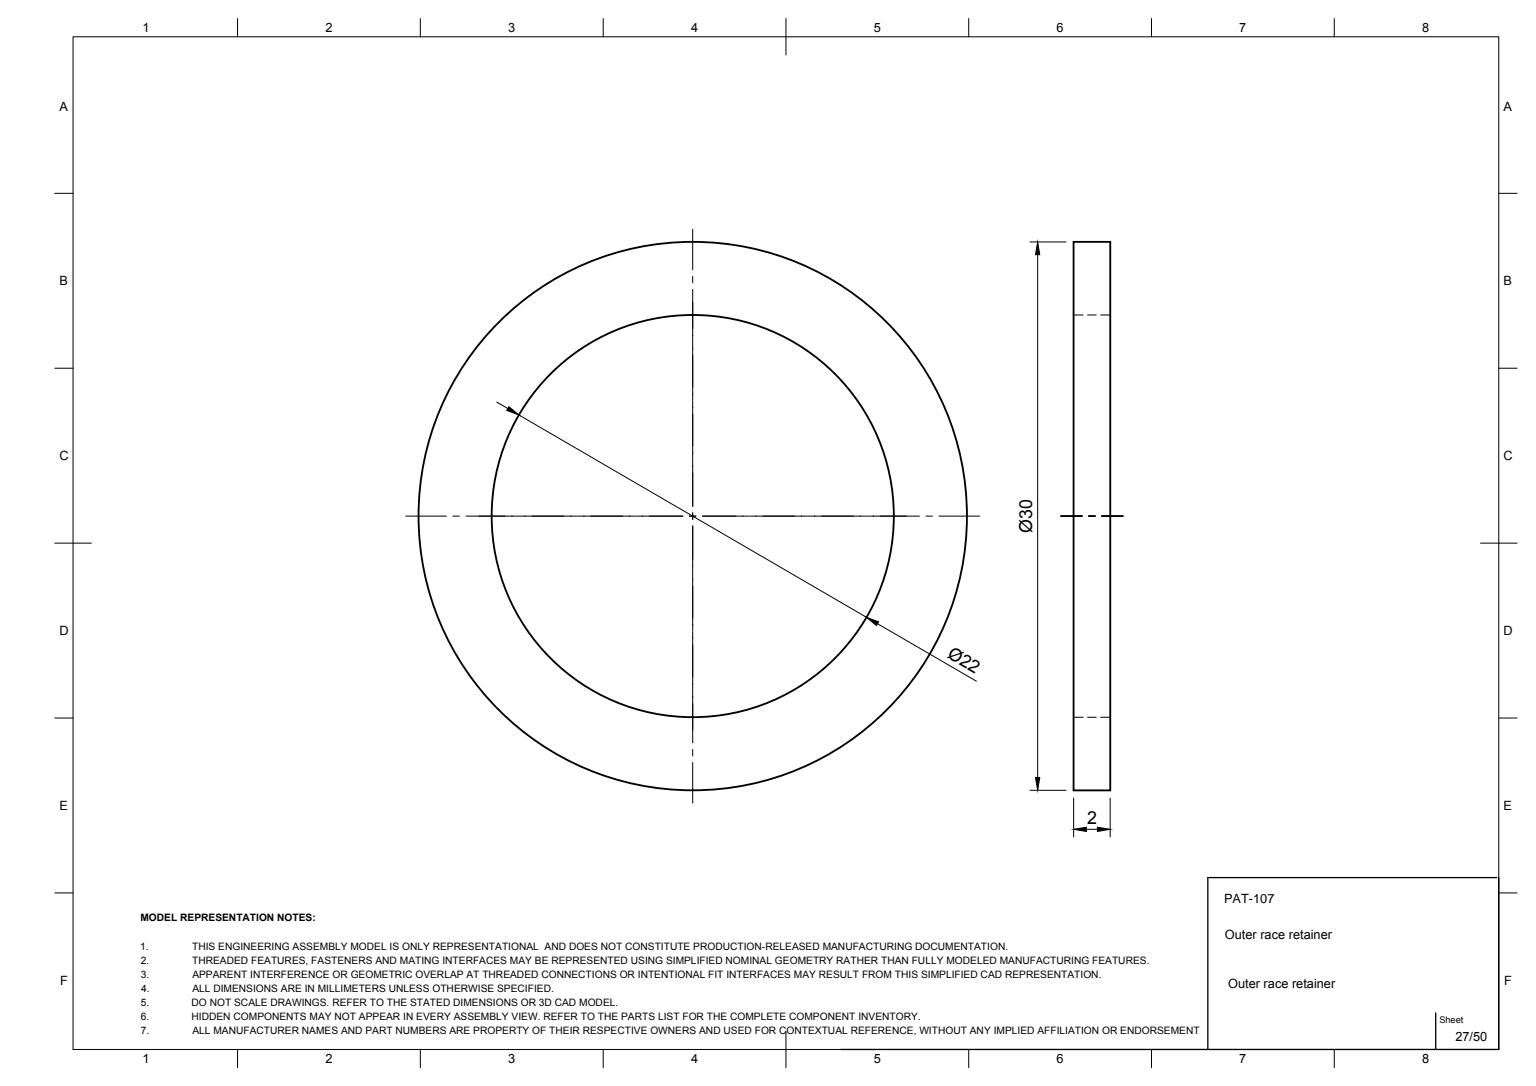
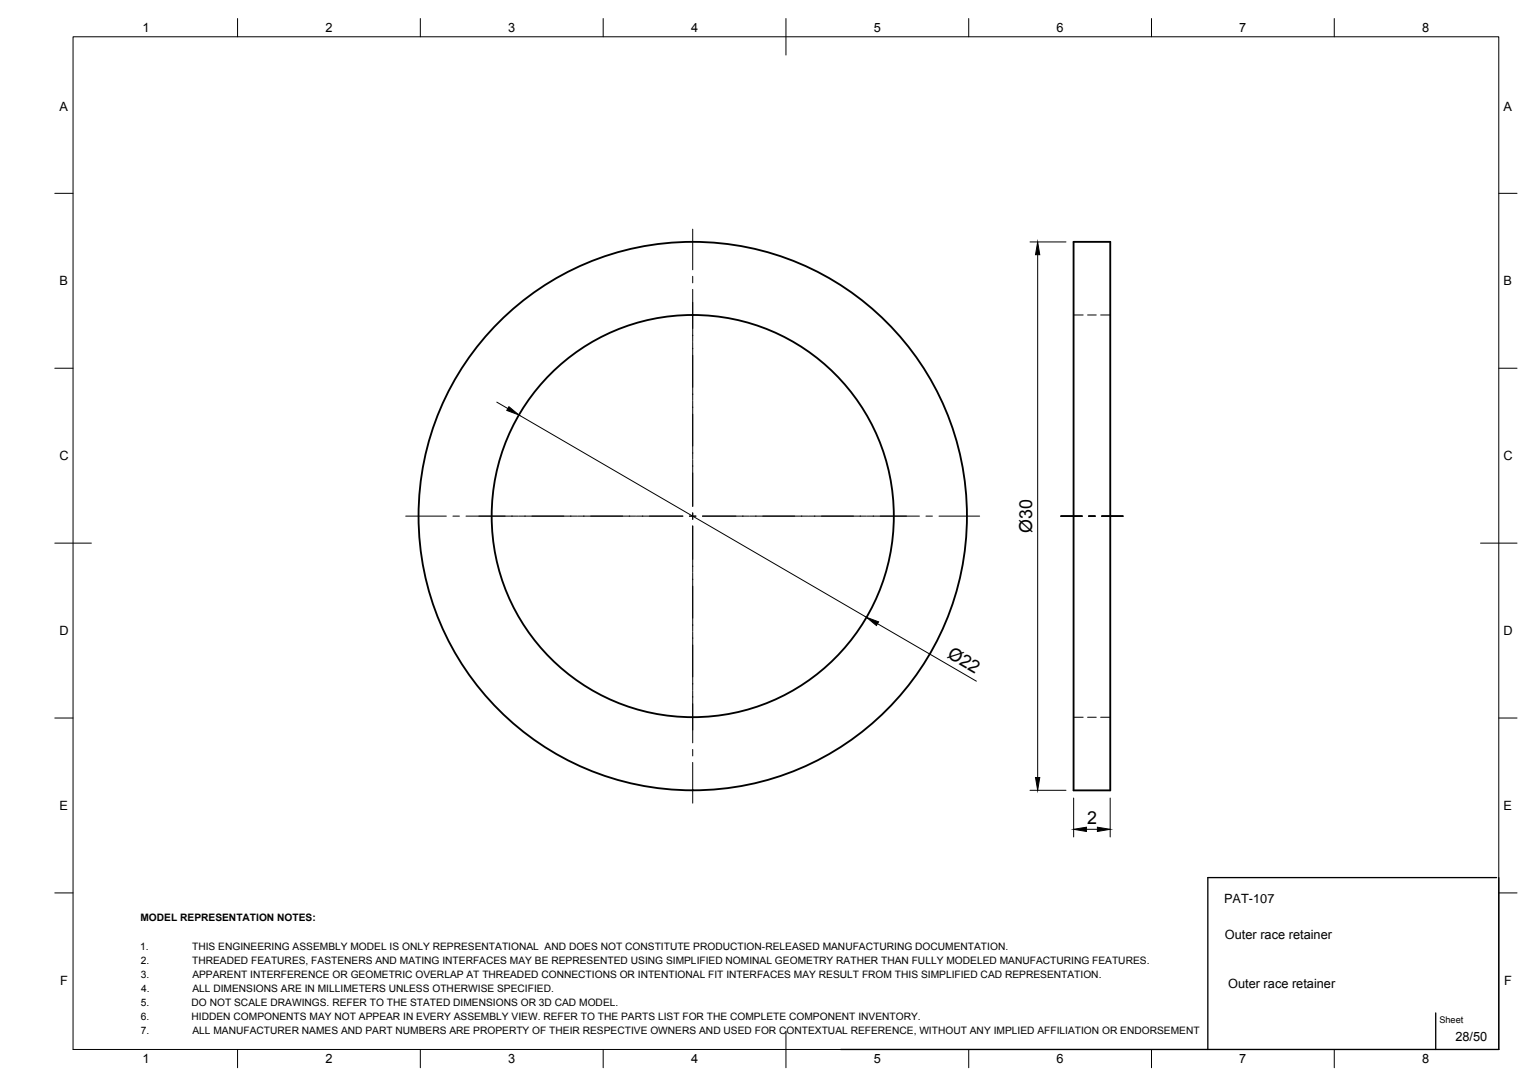
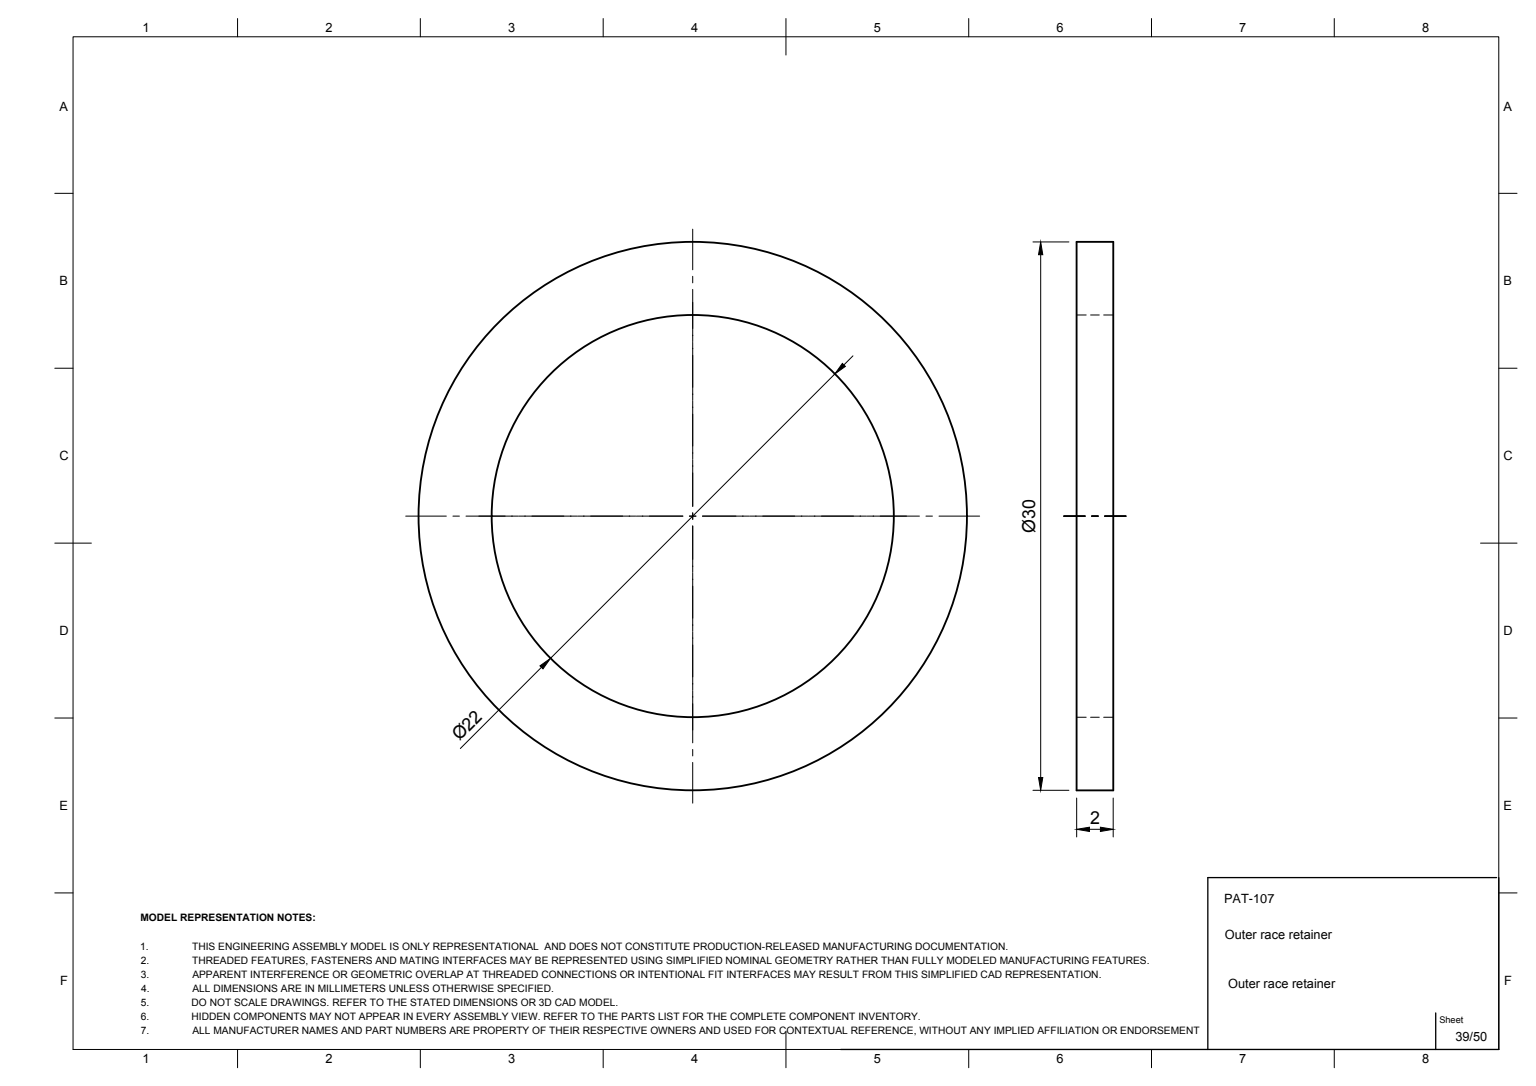
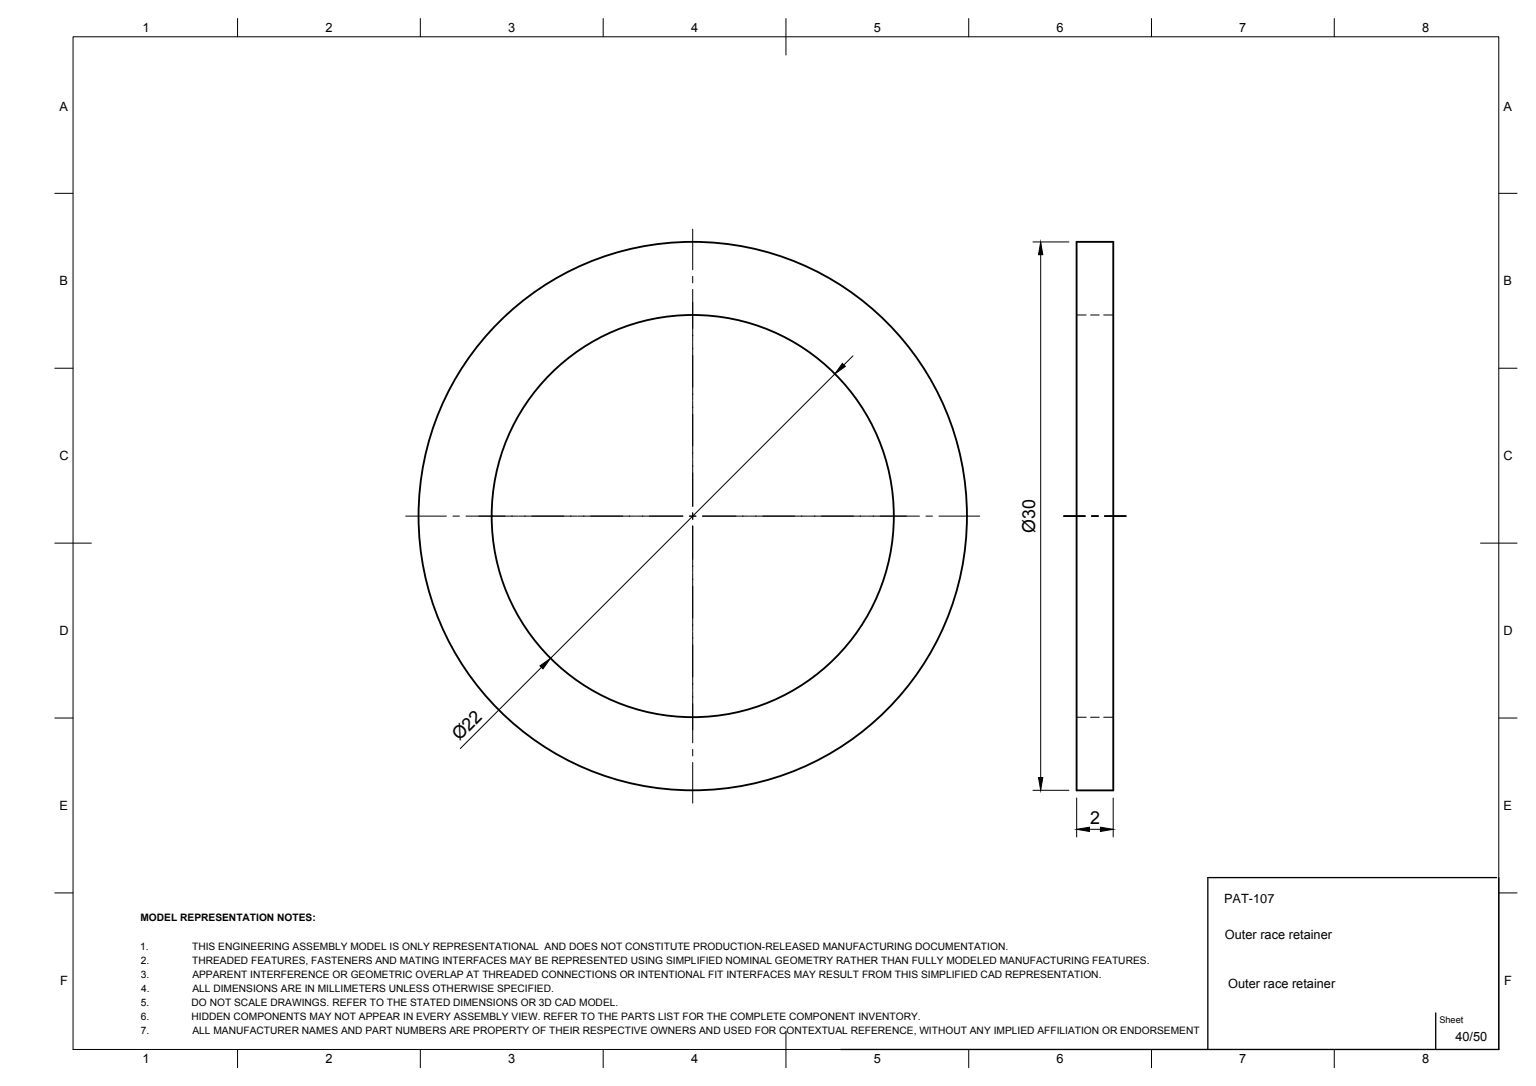
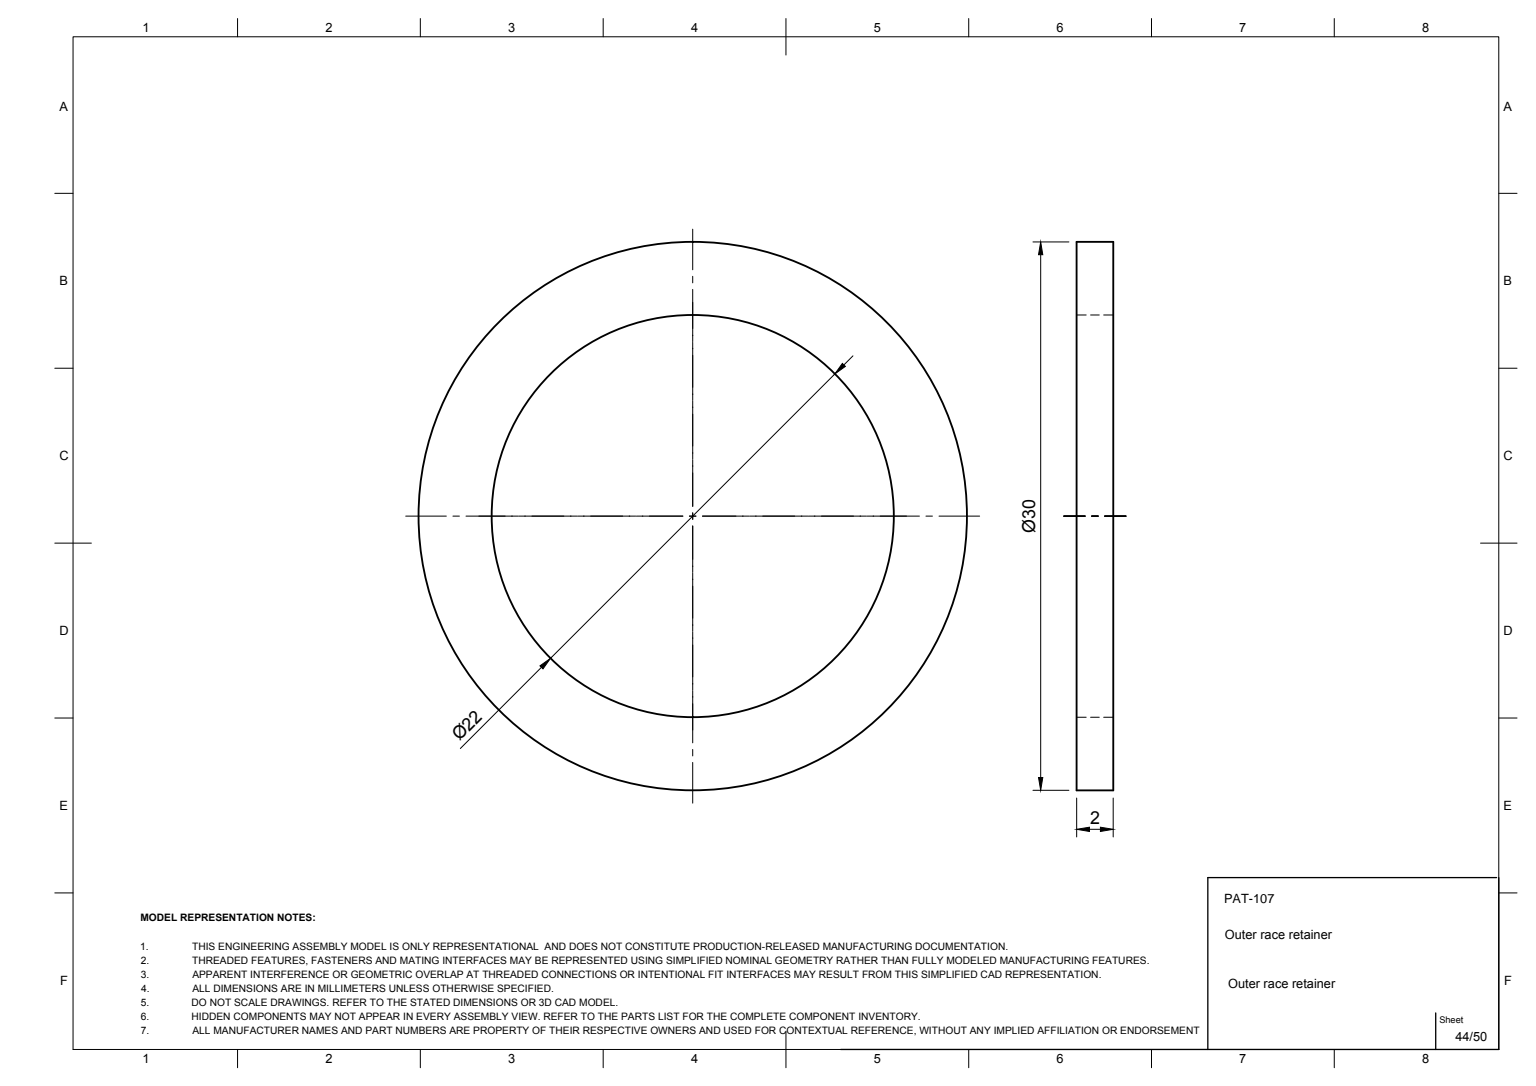
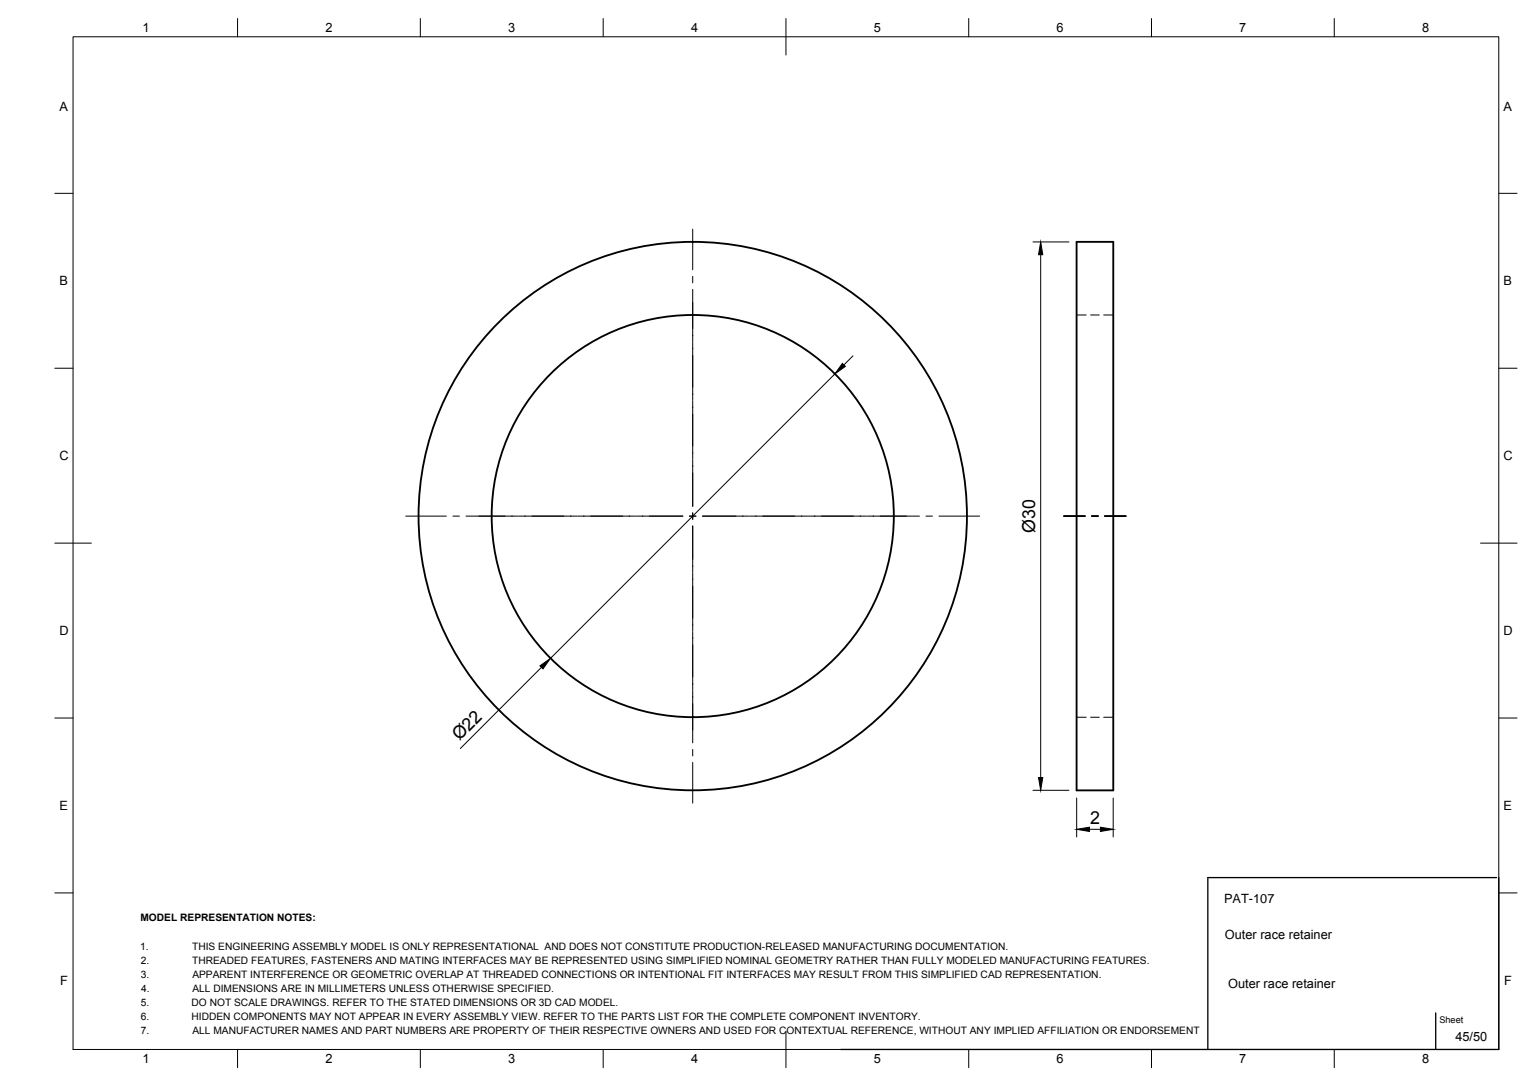
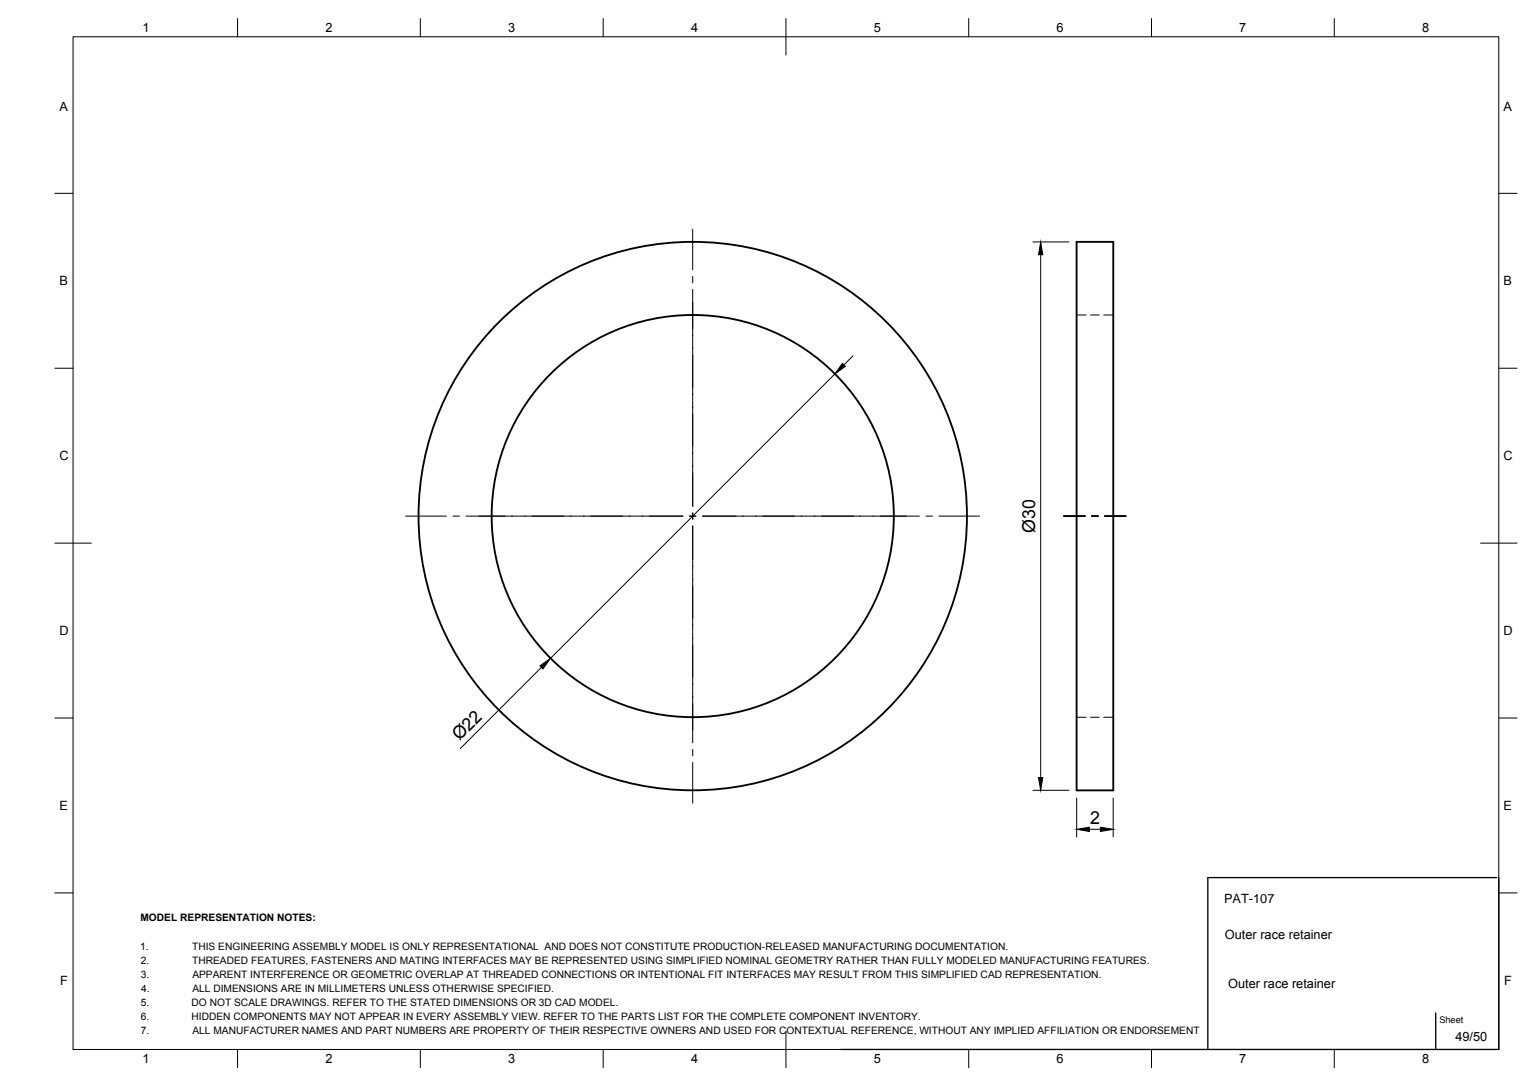
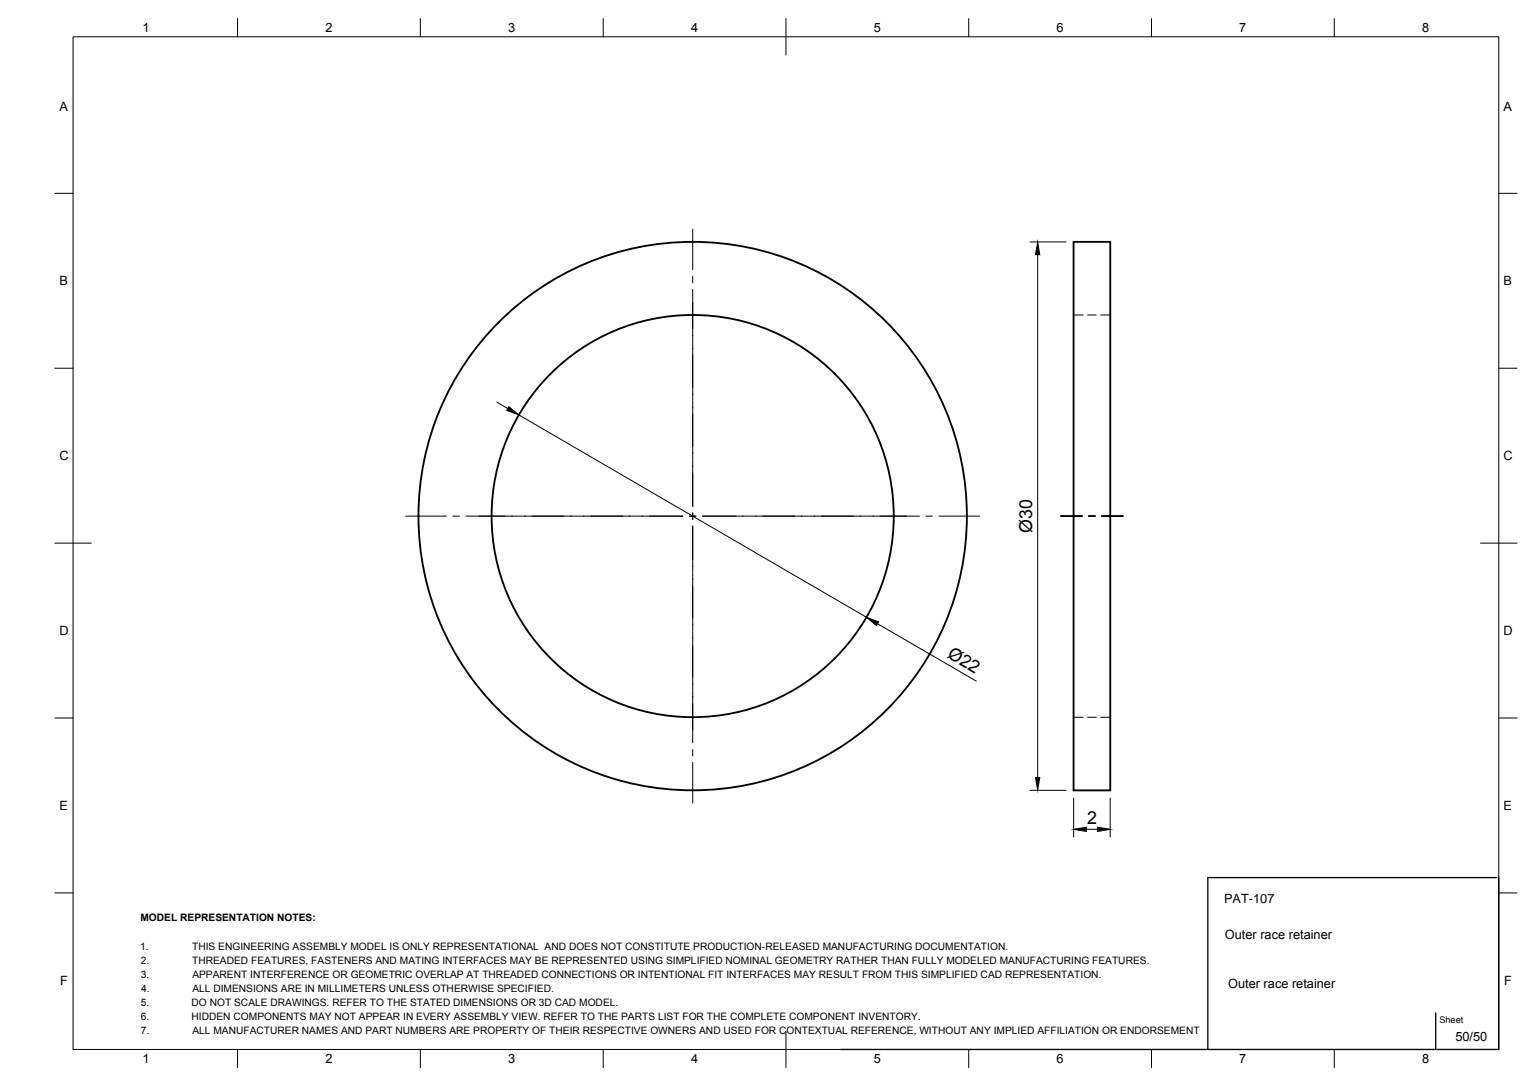
ISO-10303-21;
HEADER;
/* Generated by software containing ST-Developer
 * from STEP Tools, Inc. (www.steptools.com) 
 */

FILE_DESCRIPTION(
/* description */ ('Turntable on roller ring'),
/* implementation_level */ '2;1');

FILE_NAME(
/* name */ 'Outer race retainer.step',
/* time_stamp */ '2026-10-28T03:23:59-07:00',
/* author */ (''),
/* organization */ (''),
/* preprocessor_version */ 'ST-DEVELOPER v20.2',
/* originating_system */ 'Autodesk Translation Framework v15.17.0.0',
/* authorisation */ '');

FILE_SCHEMA (('AUTOMOTIVE_DESIGN { 1 0 10303 214 3 1 1 }'));
ENDSEC;

DATA;
#10=MECHANICAL_DESIGN_GEOMETRIC_PRESENTATION_REPRESENTATION('',(#665),#16281);
#546=SHAPE_REPRESENTATION_RELATIONSHIP('SRR','None',#16567,#601);
#601=ADVANCED_BREP_SHAPE_REPRESENTATION('',(#733),#16261);
#665=STYLED_ITEM('',(#16932),#733);
#733=MANIFOLD_SOLID_BREP('Body1',#8410);
#959=FACE_BOUND('',#2370,.T.);
#960=FACE_BOUND('',#2372,.T.);
#1211=PLANE('',#9945);
#1212=PLANE('',#9946);
#1660=FACE_OUTER_BOUND('',#2367,.T.);
#1661=FACE_OUTER_BOUND('',#2368,.T.);
#1662=FACE_OUTER_BOUND('',#2369,.T.);
#1663=FACE_OUTER_BOUND('',#2371,.T.);
#2367=EDGE_LOOP('',(#7325,#7326,#7327,#7328));
#2368=EDGE_LOOP('',(#7329,#7330,#7331,#7332));
#2369=EDGE_LOOP('',(#7333));
#2370=EDGE_LOOP('',(#7334));
#2371=EDGE_LOOP('',(#7335));
#2372=EDGE_LOOP('',(#7336));
#2938=LINE('',#15369,#3421);
#2939=LINE('',#15375,#3422);
#3421=VECTOR('',#12447,1.1);
#3422=VECTOR('',#12454,1.5);
#3833=CIRCLE('',#9940,1.1);
#3834=CIRCLE('',#9941,1.1);
#3835=CIRCLE('',#9943,1.5);
#3836=CIRCLE('',#9944,1.5);
#4509=VERTEX_POINT('',#15366);
#4510=VERTEX_POINT('',#15368);
#4511=VERTEX_POINT('',#15372);
#4512=VERTEX_POINT('',#15374);
#5473=EDGE_CURVE('',#4509,#4509,#3833,.T.);
#5474=EDGE_CURVE('',#4509,#4510,#2938,.T.);
#5475=EDGE_CURVE('',#4510,#4510,#3834,.T.);
#5476=EDGE_CURVE('',#4511,#4511,#3835,.T.);
#5477=EDGE_CURVE('',#4511,#4512,#2939,.T.);
#5478=EDGE_CURVE('',#4512,#4512,#3836,.T.);
#7325=ORIENTED_EDGE('',*,*,#5473,.F.);
#7326=ORIENTED_EDGE('',*,*,#5474,.T.);
#7327=ORIENTED_EDGE('',*,*,#5475,.T.);
#7328=ORIENTED_EDGE('',*,*,#5474,.F.);
#7329=ORIENTED_EDGE('',*,*,#5476,.F.);
#7330=ORIENTED_EDGE('',*,*,#5477,.T.);
#7331=ORIENTED_EDGE('',*,*,#5478,.T.);
#7332=ORIENTED_EDGE('',*,*,#5477,.F.);
#7333=ORIENTED_EDGE('',*,*,#5476,.T.);
#7334=ORIENTED_EDGE('',*,*,#5473,.T.);
#7335=ORIENTED_EDGE('',*,*,#5478,.F.);
#7336=ORIENTED_EDGE('',*,*,#5475,.F.);
#7819=CYLINDRICAL_SURFACE('',#9939,1.1);
#7820=CYLINDRICAL_SURFACE('',#9942,1.5);
#8263=ADVANCED_FACE('',(#1660),#7819,.F.);
#8264=ADVANCED_FACE('',(#1661),#7820,.T.);
#8265=ADVANCED_FACE('',(#1662,#959),#1211,.T.);
#8266=ADVANCED_FACE('',(#1663,#960),#1212,.F.);
#8410=CLOSED_SHELL('',(#8263,#8264,#8265,#8266));
#9938=AXIS2_PLACEMENT_3D('',#15364,#12441,#12442);
#9939=AXIS2_PLACEMENT_3D('',#15365,#12443,#12444);
#9940=AXIS2_PLACEMENT_3D('',#15367,#12445,#12446);
#9941=AXIS2_PLACEMENT_3D('',#15370,#12448,#12449);
#9942=AXIS2_PLACEMENT_3D('',#15371,#12450,#12451);
#9943=AXIS2_PLACEMENT_3D('',#15373,#12452,#12453);
#9944=AXIS2_PLACEMENT_3D('',#15376,#12455,#12456);
#9945=AXIS2_PLACEMENT_3D('',#15377,#12457,#12458);
#9946=AXIS2_PLACEMENT_3D('',#15378,#12459,#12460);
#12441=DIRECTION('axis',(0.,0.,1.));
#12442=DIRECTION('refdir',(1.,0.,0.));
#12443=DIRECTION('center_axis',(0.,1.,0.));
#12444=DIRECTION('ref_axis',(1.,0.,0.));
#12445=DIRECTION('center_axis',(0.,-1.,0.));
#12446=DIRECTION('ref_axis',(1.,0.,0.));
#12447=DIRECTION('',(0.,-1.,0.));
#12448=DIRECTION('center_axis',(0.,-1.,0.));
#12449=DIRECTION('ref_axis',(1.,0.,0.));
#12450=DIRECTION('center_axis',(0.,1.,0.));
#12451=DIRECTION('ref_axis',(1.,0.,0.));
#12452=DIRECTION('center_axis',(0.,1.,0.));
#12453=DIRECTION('ref_axis',(1.,0.,0.));
#12454=DIRECTION('',(0.,-1.,0.));
#12455=DIRECTION('center_axis',(0.,1.,0.));
#12456=DIRECTION('ref_axis',(1.,0.,0.));
#12457=DIRECTION('center_axis',(0.,1.,0.));
#12458=DIRECTION('ref_axis',(1.,0.,0.));
#12459=DIRECTION('center_axis',(0.,1.,0.));
#12460=DIRECTION('ref_axis',(1.,0.,0.));
#15364=CARTESIAN_POINT('',(0.,0.,0.));
#15365=CARTESIAN_POINT('Origin',(0.,14.35,3.5));
#15366=CARTESIAN_POINT('',(-1.1,14.55,3.5));
#15367=CARTESIAN_POINT('Origin',(0.,14.55,3.5));
#15368=CARTESIAN_POINT('',(-1.1,14.35,3.5));
#15369=CARTESIAN_POINT('',(-1.1,14.35,3.5));
#15370=CARTESIAN_POINT('Origin',(0.,14.35,3.5));
#15371=CARTESIAN_POINT('Origin',(0.,14.35,3.5));
#15372=CARTESIAN_POINT('',(-1.5,14.55,3.5));
#15373=CARTESIAN_POINT('Origin',(0.,14.55,3.5));
#15374=CARTESIAN_POINT('',(-1.5,14.35,3.5));
#15375=CARTESIAN_POINT('',(-1.5,14.35,3.5));
#15376=CARTESIAN_POINT('Origin',(0.,14.35,3.5));
#15377=CARTESIAN_POINT('Origin',(0.,14.55,3.5));
#15378=CARTESIAN_POINT('Origin',(0.,14.35,3.5));
#16192=UNCERTAINTY_MEASURE_WITH_UNIT(LENGTH_MEASURE(0.001),#16282,
'DISTANCE_ACCURACY_VALUE',
'Maximum model space distance between geometric entities at asserted c
onnectivities');
#16212=UNCERTAINTY_MEASURE_WITH_UNIT(LENGTH_MEASURE(0.001),#16282,
'DISTANCE_ACCURACY_VALUE',
'Maximum model space distance between geometric entities at asserted c
onnectivities');
#16261=(
GEOMETRIC_REPRESENTATION_CONTEXT(3)
GLOBAL_UNCERTAINTY_ASSIGNED_CONTEXT((#16192))
GLOBAL_UNIT_ASSIGNED_CONTEXT((#16282,#16284,#16285))
REPRESENTATION_CONTEXT('','3D')
);
#16281=(
GEOMETRIC_REPRESENTATION_CONTEXT(3)
GLOBAL_UNCERTAINTY_ASSIGNED_CONTEXT((#16212))
GLOBAL_UNIT_ASSIGNED_CONTEXT((#16282,#16284,#16285))
REPRESENTATION_CONTEXT('','3D')
);
#16282=(
LENGTH_UNIT()
NAMED_UNIT(*)
SI_UNIT(.CENTI.,.METRE.)
);
#16284=(
NAMED_UNIT(*)
PLANE_ANGLE_UNIT()
SI_UNIT($,.RADIAN.)
);
#16285=(
NAMED_UNIT(*)
SI_UNIT($,.STERADIAN.)
SOLID_ANGLE_UNIT()
);
#16334=SHAPE_DEFINITION_REPRESENTATION(#16468,#16567);
#16468=PRODUCT_DEFINITION_SHAPE('',$,#16636);
#16567=SHAPE_REPRESENTATION('',(#9938),#16261);
#16587=PRODUCT_DEFINITION_CONTEXT('part definition',#16793,'design');
#16636=PRODUCT_DEFINITION('Outer race retainer','Outer race retainer',#16704,
#16587);
#16704=PRODUCT_DEFINITION_FORMATION('',$,#16843);
#16793=APPLICATION_CONTEXT(
'Core Data for Automotive Mechanical Design Process');
#16794=PRODUCT_CONTEXT('part definition',#16793,'mechanical');
#16843=PRODUCT('Outer race retainer','Outer race retainer',
'Outer race retainer',(#16794));
#16926=COLOUR_RGB('Grey',0.48,0.52,0.57);
#16927=FILL_AREA_STYLE_COLOUR('',#16926);
#16928=FILL_AREA_STYLE('',(#16927));
#16929=SURFACE_STYLE_FILL_AREA(#16928);
#16930=SURFACE_SIDE_STYLE('',(#16929));
#16931=SURFACE_STYLE_USAGE(.BOTH.,#16930);
#16932=PRESENTATION_STYLE_ASSIGNMENT((#16931));
ENDSEC;
END-ISO-10303-21;
